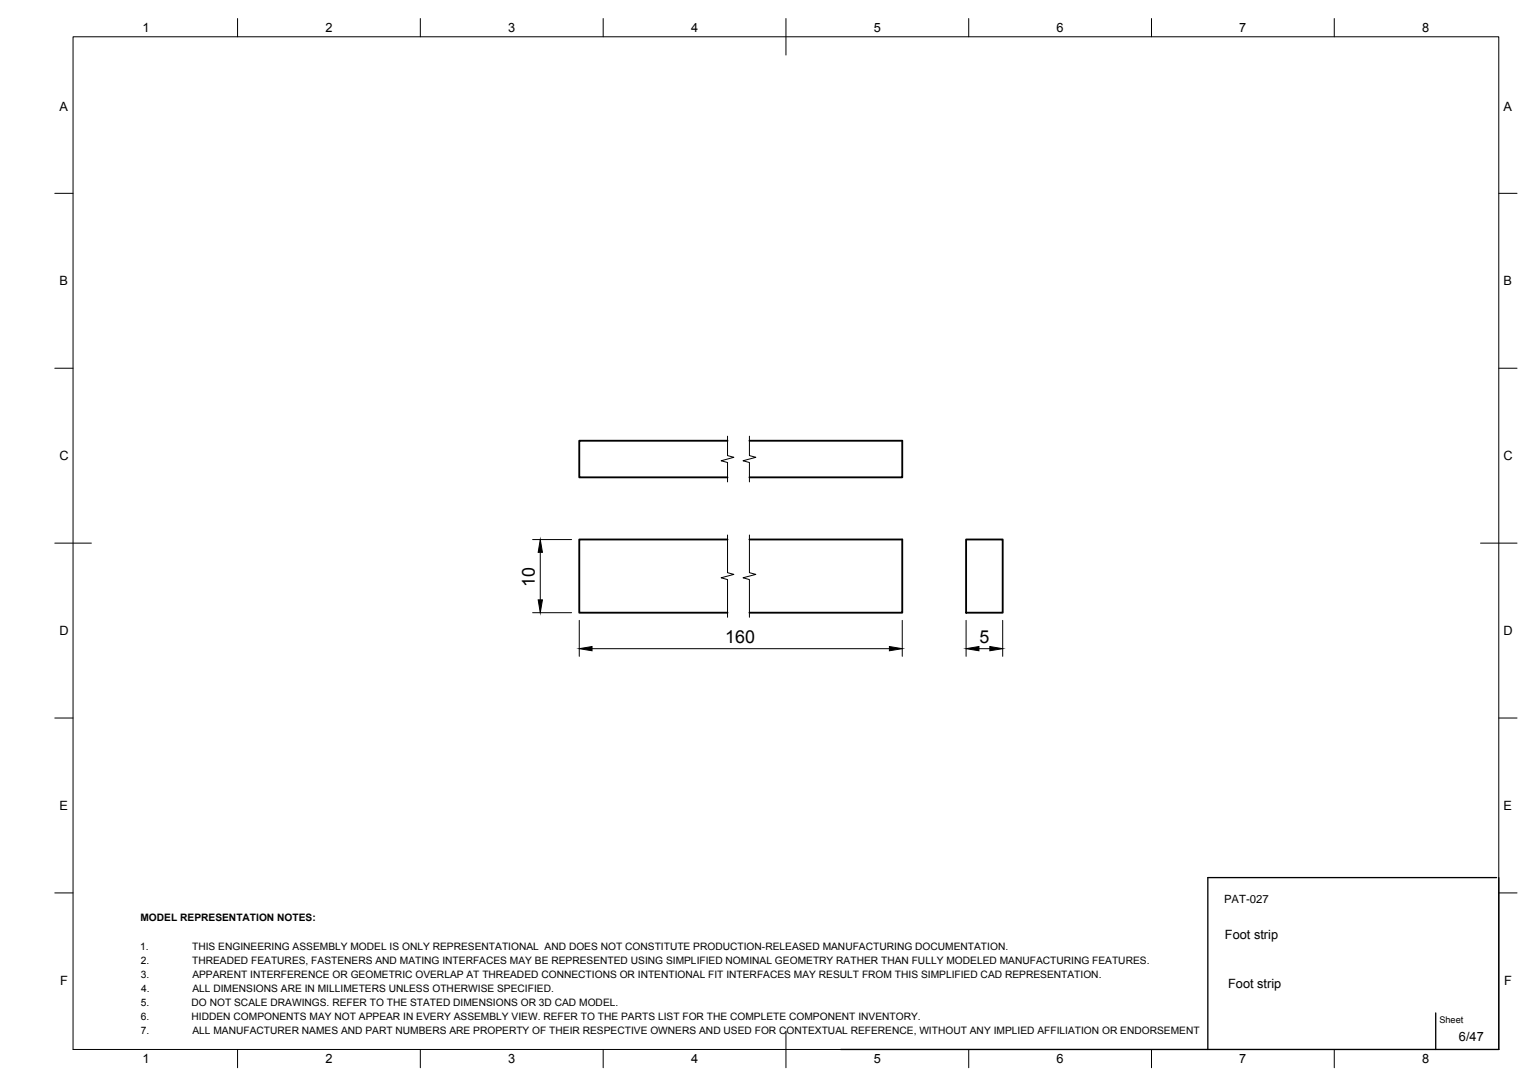
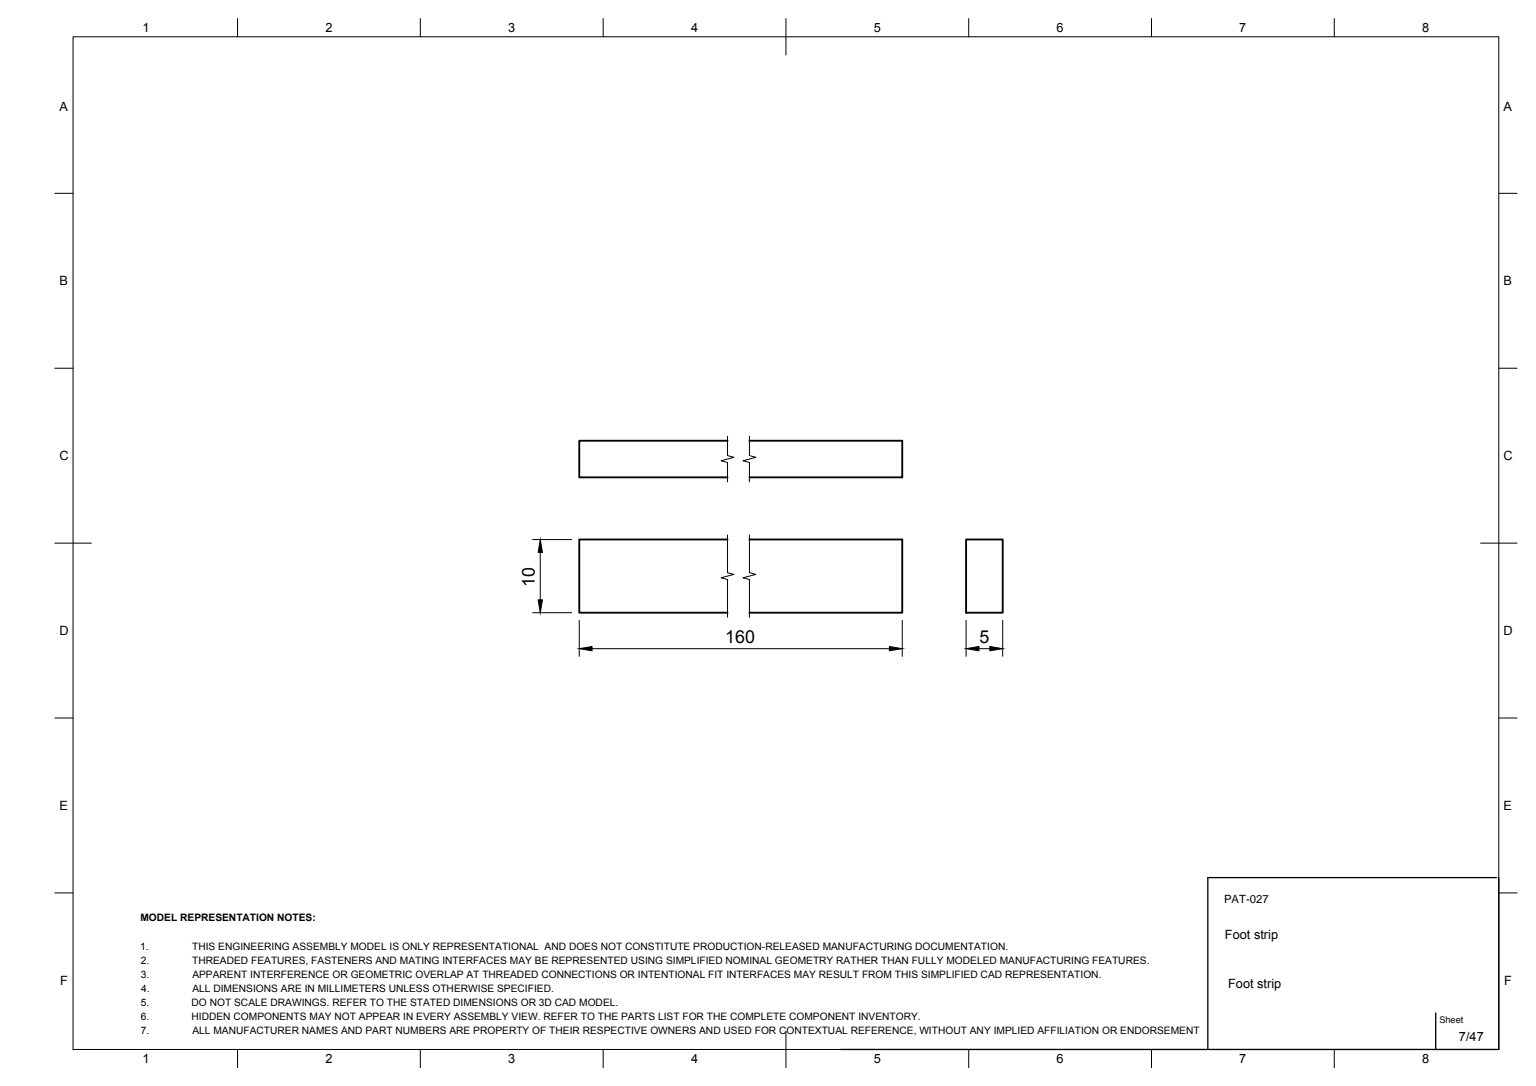
ISO-10303-21;
HEADER;
/* Generated by software containing ST-Developer
 * from STEP Tools, Inc. (www.steptools.com) 
 */

FILE_DESCRIPTION(
/* description */ ('Crank-driven oscillating fan base (mechanism only)'),

/* implementation_level */ '2;1');

FILE_NAME(
/* name */ 'Foot strip.step',
/* time_stamp */ '2026-10-28T03:25:00-07:00',
/* author */ (''),
/* organization */ (''),
/* preprocessor_version */ 'ST-DEVELOPER v20.2',
/* originating_system */ 'Autodesk Translation Framework v15.17.0.0',
/* authorisation */ '');

FILE_SCHEMA (('AUTOMOTIVE_DESIGN { 1 0 10303 214 3 1 1 }'));
ENDSEC;

DATA;
#10=MECHANICAL_DESIGN_GEOMETRIC_PRESENTATION_REPRESENTATION('',(#438),#11916);
#358=SHAPE_REPRESENTATION_RELATIONSHIP('SRR','None',#12082,#398);
#398=ADVANCED_BREP_SHAPE_REPRESENTATION('',(#486),#11873);
#438=STYLED_ITEM('',(#12361),#486);
#486=MANIFOLD_SOLID_BREP('Body1',#6068);
#698=PLANE('',#6593);
#699=PLANE('',#6594);
#700=PLANE('',#6595);
#701=PLANE('',#6596);
#702=PLANE('',#6597);
#703=PLANE('',#6598);
#900=FACE_OUTER_BOUND('',#1291,.T.);
#901=FACE_OUTER_BOUND('',#1292,.T.);
#902=FACE_OUTER_BOUND('',#1293,.T.);
#903=FACE_OUTER_BOUND('',#1294,.T.);
#904=FACE_OUTER_BOUND('',#1295,.T.);
#905=FACE_OUTER_BOUND('',#1296,.T.);
#1291=EDGE_LOOP('',(#4140,#4141,#4142,#4143));
#1292=EDGE_LOOP('',(#4144,#4145,#4146,#4147));
#1293=EDGE_LOOP('',(#4148,#4149,#4150,#4151));
#1294=EDGE_LOOP('',(#4152,#4153,#4154,#4155));
#1295=EDGE_LOOP('',(#4156,#4157,#4158,#4159));
#1296=EDGE_LOOP('',(#4160,#4161,#4162,#4163));
#1818=LINE('',#9529,#2151);
#1819=LINE('',#9531,#2152);
#1820=LINE('',#9533,#2153);
#1821=LINE('',#9534,#2154);
#1822=LINE('',#9537,#2155);
#1823=LINE('',#9539,#2156);
#1824=LINE('',#9540,#2157);
#1825=LINE('',#9543,#2158);
#1826=LINE('',#9545,#2159);
#1827=LINE('',#9546,#2160);
#1828=LINE('',#9548,#2161);
#1829=LINE('',#9549,#2162);
#2151=VECTOR('',#7501,1.);
#2152=VECTOR('',#7502,1.);
#2153=VECTOR('',#7503,1.);
#2154=VECTOR('',#7504,1.);
#2155=VECTOR('',#7507,1.);
#2156=VECTOR('',#7508,1.);
#2157=VECTOR('',#7509,1.);
#2158=VECTOR('',#7512,1.);
#2159=VECTOR('',#7513,1.);
#2160=VECTOR('',#7514,1.);
#2161=VECTOR('',#7517,1.);
#2162=VECTOR('',#7518,1.);
#2853=VERTEX_POINT('',#9527);
#2854=VERTEX_POINT('',#9528);
#2855=VERTEX_POINT('',#9530);
#2856=VERTEX_POINT('',#9532);
#2857=VERTEX_POINT('',#9536);
#2858=VERTEX_POINT('',#9538);
#2859=VERTEX_POINT('',#9542);
#2860=VERTEX_POINT('',#9544);
#3365=EDGE_CURVE('',#2853,#2854,#1818,.T.);
#3366=EDGE_CURVE('',#2854,#2855,#1819,.T.);
#3367=EDGE_CURVE('',#2856,#2855,#1820,.T.);
#3368=EDGE_CURVE('',#2853,#2856,#1821,.T.);
#3369=EDGE_CURVE('',#2857,#2853,#1822,.T.);
#3370=EDGE_CURVE('',#2858,#2856,#1823,.T.);
#3371=EDGE_CURVE('',#2857,#2858,#1824,.T.);
#3372=EDGE_CURVE('',#2859,#2857,#1825,.T.);
#3373=EDGE_CURVE('',#2860,#2858,#1826,.T.);
#3374=EDGE_CURVE('',#2859,#2860,#1827,.T.);
#3375=EDGE_CURVE('',#2854,#2859,#1828,.T.);
#3376=EDGE_CURVE('',#2855,#2860,#1829,.T.);
#4140=ORIENTED_EDGE('',*,*,#3365,.T.);
#4141=ORIENTED_EDGE('',*,*,#3366,.T.);
#4142=ORIENTED_EDGE('',*,*,#3367,.F.);
#4143=ORIENTED_EDGE('',*,*,#3368,.F.);
#4144=ORIENTED_EDGE('',*,*,#3369,.T.);
#4145=ORIENTED_EDGE('',*,*,#3368,.T.);
#4146=ORIENTED_EDGE('',*,*,#3370,.F.);
#4147=ORIENTED_EDGE('',*,*,#3371,.F.);
#4148=ORIENTED_EDGE('',*,*,#3372,.T.);
#4149=ORIENTED_EDGE('',*,*,#3371,.T.);
#4150=ORIENTED_EDGE('',*,*,#3373,.F.);
#4151=ORIENTED_EDGE('',*,*,#3374,.F.);
#4152=ORIENTED_EDGE('',*,*,#3375,.T.);
#4153=ORIENTED_EDGE('',*,*,#3374,.T.);
#4154=ORIENTED_EDGE('',*,*,#3376,.F.);
#4155=ORIENTED_EDGE('',*,*,#3366,.F.);
#4156=ORIENTED_EDGE('',*,*,#3376,.T.);
#4157=ORIENTED_EDGE('',*,*,#3373,.T.);
#4158=ORIENTED_EDGE('',*,*,#3370,.T.);
#4159=ORIENTED_EDGE('',*,*,#3367,.T.);
#4160=ORIENTED_EDGE('',*,*,#3375,.F.);
#4161=ORIENTED_EDGE('',*,*,#3365,.F.);
#4162=ORIENTED_EDGE('',*,*,#3369,.F.);
#4163=ORIENTED_EDGE('',*,*,#3372,.F.);
#5706=ADVANCED_FACE('',(#900),#698,.T.);
#5707=ADVANCED_FACE('',(#901),#699,.T.);
#5708=ADVANCED_FACE('',(#902),#700,.T.);
#5709=ADVANCED_FACE('',(#903),#701,.T.);
#5710=ADVANCED_FACE('',(#904),#702,.T.);
#5711=ADVANCED_FACE('',(#905),#703,.F.);
#6068=CLOSED_SHELL('',(#5706,#5707,#5708,#5709,#5710,#5711));
#6592=AXIS2_PLACEMENT_3D('',#9525,#7497,#7498);
#6593=AXIS2_PLACEMENT_3D('',#9526,#7499,#7500);
#6594=AXIS2_PLACEMENT_3D('',#9535,#7505,#7506);
#6595=AXIS2_PLACEMENT_3D('',#9541,#7510,#7511);
#6596=AXIS2_PLACEMENT_3D('',#9547,#7515,#7516);
#6597=AXIS2_PLACEMENT_3D('',#9550,#7519,#7520);
#6598=AXIS2_PLACEMENT_3D('',#9551,#7521,#7522);
#7497=DIRECTION('axis',(0.,0.,1.));
#7498=DIRECTION('refdir',(1.,0.,0.));
#7499=DIRECTION('center_axis',(0.,1.,0.));
#7500=DIRECTION('ref_axis',(-1.,0.,0.));
#7501=DIRECTION('',(-1.,0.,0.));
#7502=DIRECTION('',(0.,0.,1.));
#7503=DIRECTION('',(-1.,0.,0.));
#7504=DIRECTION('',(0.,0.,1.));
#7505=DIRECTION('center_axis',(1.,0.,0.));
#7506=DIRECTION('ref_axis',(0.,1.,0.));
#7507=DIRECTION('',(0.,1.,0.));
#7508=DIRECTION('',(0.,1.,0.));
#7509=DIRECTION('',(0.,0.,1.));
#7510=DIRECTION('center_axis',(0.,-1.,0.));
#7511=DIRECTION('ref_axis',(1.,0.,0.));
#7512=DIRECTION('',(1.,0.,0.));
#7513=DIRECTION('',(1.,0.,0.));
#7514=DIRECTION('',(0.,0.,1.));
#7515=DIRECTION('center_axis',(-1.,0.,0.));
#7516=DIRECTION('ref_axis',(0.,-1.,0.));
#7517=DIRECTION('',(0.,-1.,0.));
#7518=DIRECTION('',(0.,-1.,0.));
#7519=DIRECTION('center_axis',(0.,0.,1.));
#7520=DIRECTION('ref_axis',(1.,0.,0.));
#7521=DIRECTION('center_axis',(0.,0.,1.));
#7522=DIRECTION('ref_axis',(1.,0.,0.));
#9525=CARTESIAN_POINT('',(0.,0.,0.));
#9526=CARTESIAN_POINT('Origin',(12.,-3.,-0.5));
#9527=CARTESIAN_POINT('',(12.,-3.,-0.5));
#9528=CARTESIAN_POINT('',(-4.,-3.,-0.5));
#9529=CARTESIAN_POINT('',(12.,-3.,-0.5));
#9530=CARTESIAN_POINT('',(-4.,-3.,0.));
#9531=CARTESIAN_POINT('',(-4.,-3.,-0.5));
#9532=CARTESIAN_POINT('',(12.,-3.,0.));
#9533=CARTESIAN_POINT('',(12.,-3.,0.));
#9534=CARTESIAN_POINT('',(12.,-3.,-0.5));
#9535=CARTESIAN_POINT('Origin',(12.,-4.,-0.5));
#9536=CARTESIAN_POINT('',(12.,-4.,-0.5));
#9537=CARTESIAN_POINT('',(12.,-4.,-0.5));
#9538=CARTESIAN_POINT('',(12.,-4.,0.));
#9539=CARTESIAN_POINT('',(12.,-4.,0.));
#9540=CARTESIAN_POINT('',(12.,-4.,-0.5));
#9541=CARTESIAN_POINT('Origin',(-4.,-4.,-0.5));
#9542=CARTESIAN_POINT('',(-4.,-4.,-0.5));
#9543=CARTESIAN_POINT('',(-4.,-4.,-0.5));
#9544=CARTESIAN_POINT('',(-4.,-4.,0.));
#9545=CARTESIAN_POINT('',(-4.,-4.,0.));
#9546=CARTESIAN_POINT('',(-4.,-4.,-0.5));
#9547=CARTESIAN_POINT('Origin',(-4.,-3.,-0.5));
#9548=CARTESIAN_POINT('',(-4.,-3.,-0.5));
#9549=CARTESIAN_POINT('',(-4.,-3.,0.));
#9550=CARTESIAN_POINT('Origin',(4.,-3.5,0.));
#9551=CARTESIAN_POINT('Origin',(4.,-3.5,-0.5));
#11826=UNCERTAINTY_MEASURE_WITH_UNIT(LENGTH_MEASURE(0.001),#11917,
'DISTANCE_ACCURACY_VALUE',
'Maximum model space distance between geometric entities at asserted c
onnectivities');
#11869=UNCERTAINTY_MEASURE_WITH_UNIT(LENGTH_MEASURE(0.001),#11917,
'DISTANCE_ACCURACY_VALUE',
'Maximum model space distance between geometric entities at asserted c
onnectivities');
#11873=(
GEOMETRIC_REPRESENTATION_CONTEXT(3)
GLOBAL_UNCERTAINTY_ASSIGNED_CONTEXT((#11826))
GLOBAL_UNIT_ASSIGNED_CONTEXT((#11917,#11919,#11920))
REPRESENTATION_CONTEXT('','3D')
);
#11916=(
GEOMETRIC_REPRESENTATION_CONTEXT(3)
GLOBAL_UNCERTAINTY_ASSIGNED_CONTEXT((#11869))
GLOBAL_UNIT_ASSIGNED_CONTEXT((#11917,#11919,#11920))
REPRESENTATION_CONTEXT('','3D')
);
#11917=(
LENGTH_UNIT()
NAMED_UNIT(*)
SI_UNIT(.CENTI.,.METRE.)
);
#11919=(
NAMED_UNIT(*)
PLANE_ANGLE_UNIT()
SI_UNIT($,.RADIAN.)
);
#11920=(
NAMED_UNIT(*)
SI_UNIT($,.STERADIAN.)
SOLID_ANGLE_UNIT()
);
#11924=SHAPE_DEFINITION_REPRESENTATION(#11970,#12082);
#11970=PRODUCT_DEFINITION_SHAPE('',$,#12129);
#12082=SHAPE_REPRESENTATION('',(#6592),#11873);
#12125=PRODUCT_DEFINITION_CONTEXT('part definition',#12265,'design');
#12129=PRODUCT_DEFINITION('Foot strip','Foot strip',#12175,#12125);
#12175=PRODUCT_DEFINITION_FORMATION('',$,#12270);
#12265=APPLICATION_CONTEXT(
'Core Data for Automotive Mechanical Design Process');
#12266=PRODUCT_CONTEXT('part definition',#12265,'mechanical');
#12270=PRODUCT('Foot strip','Foot strip','Foot strip',(#12266));
#12355=COLOUR_RGB('Light Blue',0.38,0.62,0.78);
#12356=FILL_AREA_STYLE_COLOUR('',#12355);
#12357=FILL_AREA_STYLE('',(#12356));
#12358=SURFACE_STYLE_FILL_AREA(#12357);
#12359=SURFACE_SIDE_STYLE('',(#12358));
#12360=SURFACE_STYLE_USAGE(.BOTH.,#12359);
#12361=PRESENTATION_STYLE_ASSIGNMENT((#12360));
ENDSEC;
END-ISO-10303-21;
